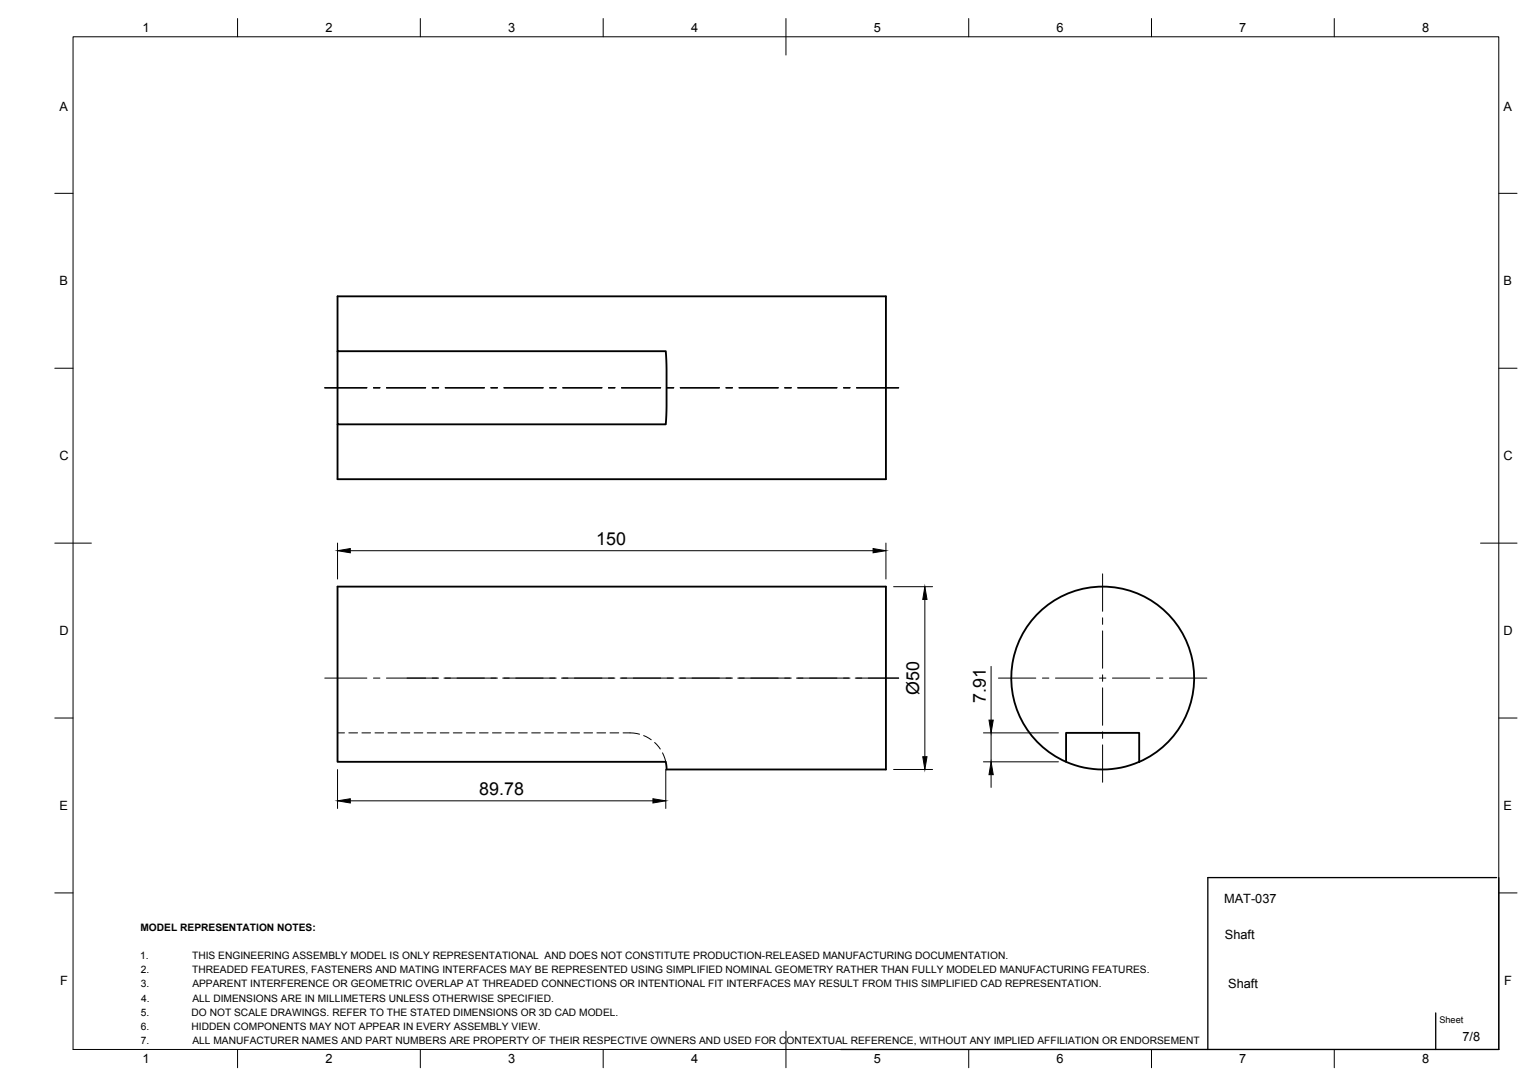
ISO-10303-21;
HEADER;
/* Generated by software containing ST-Developer
 * from STEP Tools, Inc. (www.steptools.com) 
 */

FILE_DESCRIPTION(
/* description */ ('STEP AP214'),
/* implementation_level */ '2;1');

FILE_NAME(
/* name */ 'shaft.step',
/* time_stamp */ '2026-11-14T21:09:07-08:00',
/* author */ (''),
/* organization */ (''),
/* preprocessor_version */ 'ST-DEVELOPER v20.2',
/* originating_system */ 'Autodesk Translation Framework v15.17.0.0',
/* authorisation */ '');

FILE_SCHEMA (('AUTOMOTIVE_DESIGN { 1 0 10303 214 3 1 1 }'));
ENDSEC;

DATA;
#10=MECHANICAL_DESIGN_GEOMETRIC_PRESENTATION_REPRESENTATION('',(#83),#2059);
#69=SHAPE_REPRESENTATION_RELATIONSHIP('SRR','None',#2099,#76);
#76=ADVANCED_BREP_SHAPE_REPRESENTATION('',(#90),#2057);
#83=STYLED_ITEM('',(#2142),#90);
#90=MANIFOLD_SOLID_BREP('Body1',#980);
#116=PLANE('',#1148);
#117=PLANE('',#1149);
#118=PLANE('',#1150);
#119=PLANE('',#1152);
#120=PLANE('',#1154);
#155=B_SPLINE_CURVE_WITH_KNOTS('',3,(#1969,#1970,#1971,#1972,#1973,#1974,
#1975,#1976,#1977,#1978,#1979,#1980,#1981,#1982),.UNSPECIFIED.,.F.,.F.,
(4,2,2,2,2,2,4),(-3.67157631505784,-3.33396300865433,-3.01698728047981,
-2.7000115523053,-2.38303582413079,-2.06606009595627,-1.72844678955265),
 .UNSPECIFIED.);
#199=FACE_OUTER_BOUND('',#275,.T.);
#200=FACE_OUTER_BOUND('',#276,.T.);
#201=FACE_OUTER_BOUND('',#277,.T.);
#202=FACE_OUTER_BOUND('',#278,.T.);
#203=FACE_OUTER_BOUND('',#279,.T.);
#204=FACE_OUTER_BOUND('',#280,.T.);
#205=FACE_OUTER_BOUND('',#281,.T.);
#275=EDGE_LOOP('',(#843,#844,#845,#846,#847,#848,#849,#850));
#276=EDGE_LOOP('',(#851,#852,#853,#854,#855));
#277=EDGE_LOOP('',(#856));
#278=EDGE_LOOP('',(#857,#858,#859,#860));
#279=EDGE_LOOP('',(#861,#862,#863,#864));
#280=EDGE_LOOP('',(#865,#866,#867,#868));
#281=EDGE_LOOP('',(#869,#870,#871,#872));
#336=LINE('',#1962,#401);
#337=LINE('',#1967,#402);
#338=LINE('',#1983,#403);
#339=LINE('',#1986,#404);
#340=LINE('',#1988,#405);
#341=LINE('',#1989,#406);
#342=LINE('',#1994,#407);
#343=LINE('',#1997,#408);
#344=LINE('',#2000,#409);
#401=VECTOR('',#1400,25.0000000000002);
#402=VECTOR('',#1405,1000.);
#403=VECTOR('',#1406,1000.);
#404=VECTOR('',#1409,1000.);
#405=VECTOR('',#1410,1000.);
#406=VECTOR('',#1411,1000.);
#407=VECTOR('',#1418,1000.);
#408=VECTOR('',#1421,1000.);
#409=VECTOR('',#1426,1000.);
#452=CIRCLE('',#1145,25.0000000000002);
#453=CIRCLE('',#1146,25.0000000000002);
#454=CIRCLE('',#1147,25.0000000000002);
#455=CIRCLE('',#1151,10.0000000000001);
#456=CIRCLE('',#1153,10.0000000000001);
#522=VERTEX_POINT('',#1958);
#523=VERTEX_POINT('',#1959);
#524=VERTEX_POINT('',#1961);
#525=VERTEX_POINT('',#1964);
#526=VERTEX_POINT('',#1966);
#527=VERTEX_POINT('',#1968);
#528=VERTEX_POINT('',#1985);
#529=VERTEX_POINT('',#1987);
#530=VERTEX_POINT('',#1992);
#531=VERTEX_POINT('',#1996);
#632=EDGE_CURVE('',#522,#523,#452,.T.);
#633=EDGE_CURVE('',#523,#524,#336,.T.);
#634=EDGE_CURVE('',#524,#524,#453,.T.);
#635=EDGE_CURVE('',#523,#525,#454,.T.);
#636=EDGE_CURVE('',#526,#525,#337,.T.);
#637=EDGE_CURVE('',#526,#527,#155,.T.);
#638=EDGE_CURVE('',#522,#527,#338,.T.);
#639=EDGE_CURVE('',#528,#522,#339,.T.);
#640=EDGE_CURVE('',#528,#529,#340,.T.);
#641=EDGE_CURVE('',#529,#525,#341,.T.);
#642=EDGE_CURVE('',#527,#530,#455,.T.);
#643=EDGE_CURVE('',#530,#528,#342,.T.);
#644=EDGE_CURVE('',#531,#529,#343,.T.);
#645=EDGE_CURVE('',#531,#526,#456,.T.);
#646=EDGE_CURVE('',#530,#531,#344,.T.);
#843=ORIENTED_EDGE('',*,*,#632,.T.);
#844=ORIENTED_EDGE('',*,*,#633,.T.);
#845=ORIENTED_EDGE('',*,*,#634,.F.);
#846=ORIENTED_EDGE('',*,*,#633,.F.);
#847=ORIENTED_EDGE('',*,*,#635,.T.);
#848=ORIENTED_EDGE('',*,*,#636,.F.);
#849=ORIENTED_EDGE('',*,*,#637,.T.);
#850=ORIENTED_EDGE('',*,*,#638,.F.);
#851=ORIENTED_EDGE('',*,*,#639,.F.);
#852=ORIENTED_EDGE('',*,*,#640,.T.);
#853=ORIENTED_EDGE('',*,*,#641,.T.);
#854=ORIENTED_EDGE('',*,*,#635,.F.);
#855=ORIENTED_EDGE('',*,*,#632,.F.);
#856=ORIENTED_EDGE('',*,*,#634,.T.);
#857=ORIENTED_EDGE('',*,*,#638,.T.);
#858=ORIENTED_EDGE('',*,*,#642,.T.);
#859=ORIENTED_EDGE('',*,*,#643,.T.);
#860=ORIENTED_EDGE('',*,*,#639,.T.);
#861=ORIENTED_EDGE('',*,*,#644,.F.);
#862=ORIENTED_EDGE('',*,*,#645,.T.);
#863=ORIENTED_EDGE('',*,*,#636,.T.);
#864=ORIENTED_EDGE('',*,*,#641,.F.);
#865=ORIENTED_EDGE('',*,*,#643,.F.);
#866=ORIENTED_EDGE('',*,*,#646,.T.);
#867=ORIENTED_EDGE('',*,*,#644,.T.);
#868=ORIENTED_EDGE('',*,*,#640,.F.);
#869=ORIENTED_EDGE('',*,*,#642,.F.);
#870=ORIENTED_EDGE('',*,*,#637,.F.);
#871=ORIENTED_EDGE('',*,*,#645,.F.);
#872=ORIENTED_EDGE('',*,*,#646,.F.);
#915=CYLINDRICAL_SURFACE('',#1144,25.0000000000002);
#916=CYLINDRICAL_SURFACE('',#1155,10.0000000000001);
#962=ADVANCED_FACE('',(#199),#915,.T.);
#963=ADVANCED_FACE('',(#200),#116,.F.);
#964=ADVANCED_FACE('',(#201),#117,.T.);
#965=ADVANCED_FACE('',(#202),#118,.T.);
#966=ADVANCED_FACE('',(#203),#119,.T.);
#967=ADVANCED_FACE('',(#204),#120,.T.);
#968=ADVANCED_FACE('',(#205),#916,.F.);
#980=CLOSED_SHELL('',(#962,#963,#964,#965,#966,#967,#968));
#1143=AXIS2_PLACEMENT_3D('',#1956,#1394,#1395);
#1144=AXIS2_PLACEMENT_3D('',#1957,#1396,#1397);
#1145=AXIS2_PLACEMENT_3D('',#1960,#1398,#1399);
#1146=AXIS2_PLACEMENT_3D('',#1963,#1401,#1402);
#1147=AXIS2_PLACEMENT_3D('',#1965,#1403,#1404);
#1148=AXIS2_PLACEMENT_3D('',#1984,#1407,#1408);
#1149=AXIS2_PLACEMENT_3D('',#1990,#1412,#1413);
#1150=AXIS2_PLACEMENT_3D('',#1991,#1414,#1415);
#1151=AXIS2_PLACEMENT_3D('',#1993,#1416,#1417);
#1152=AXIS2_PLACEMENT_3D('',#1995,#1419,#1420);
#1153=AXIS2_PLACEMENT_3D('',#1998,#1422,#1423);
#1154=AXIS2_PLACEMENT_3D('',#1999,#1424,#1425);
#1155=AXIS2_PLACEMENT_3D('',#2001,#1427,#1428);
#1394=DIRECTION('axis',(0.,0.,1.));
#1395=DIRECTION('refdir',(1.,0.,0.));
#1396=DIRECTION('center_axis',(1.40946282423116E-17,-7.79000143905744E-30,
-1.));
#1397=DIRECTION('ref_axis',(-1.,1.65167752030648E-30,-1.40946282423116E-17));
#1398=DIRECTION('center_axis',(-1.40946282423116E-17,7.79000143905744E-30,
1.));
#1399=DIRECTION('ref_axis',(1.,-1.65167752030648E-30,1.40946282423116E-17));
#1400=DIRECTION('',(-1.40946282423116E-17,7.79000143905744E-30,1.));
#1401=DIRECTION('center_axis',(-1.40946282423116E-17,7.79000143905744E-30,
1.));
#1402=DIRECTION('ref_axis',(1.,-1.65167752030648E-30,1.40946282423116E-17));
#1403=DIRECTION('center_axis',(-1.40946282423116E-17,7.79000143905744E-30,
1.));
#1404=DIRECTION('ref_axis',(1.,-1.65167752030648E-30,1.40946282423116E-17));
#1405=DIRECTION('',(1.40946282423116E-17,-7.79000143905744E-30,-1.));
#1406=DIRECTION('',(-1.40946282423116E-17,7.79000143905744E-30,1.));
#1407=DIRECTION('center_axis',(-1.40946282423114E-17,7.79000143905744E-30,
1.));
#1408=DIRECTION('ref_axis',(1.,-1.65167752030648E-30,1.40946282423114E-17));
#1409=DIRECTION('',(-1.84889274661175E-30,1.,7.29696337329436E-30));
#1410=DIRECTION('',(1.,-1.65167752030648E-30,1.40946282423114E-17));
#1411=DIRECTION('',(-1.84889274661175E-30,1.,7.29696337329436E-30));
#1412=DIRECTION('center_axis',(-1.40946282423114E-17,7.79000143905744E-30,
1.));
#1413=DIRECTION('ref_axis',(1.,-1.65167752030648E-30,1.40946282423114E-17));
#1414=DIRECTION('center_axis',(1.,-1.7009813268828E-30,1.40946282423116E-17));
#1415=DIRECTION('ref_axis',(1.40946282423116E-17,-7.79000143905744E-30,
-1.));
#1416=DIRECTION('center_axis',(1.,-1.7009813268828E-30,1.04083408558607E-17));
#1417=DIRECTION('ref_axis',(1.04083408558607E-17,-1.77043934396503E-47,
-1.));
#1418=DIRECTION('',(1.04083408558609E-17,-7.69139382590482E-30,-1.));
#1419=DIRECTION('center_axis',(-1.,1.7009813268828E-30,-1.40946282423116E-17));
#1420=DIRECTION('ref_axis',(-1.40946282423116E-17,7.79000143905744E-30,
1.));
#1421=DIRECTION('',(1.04083408558609E-17,-7.69139382590482E-30,-1.));
#1422=DIRECTION('center_axis',(-1.,1.7009813268828E-30,-1.04083408558607E-17));
#1423=DIRECTION('ref_axis',(-1.04083408558607E-17,1.77043934396503E-47,
1.));
#1424=DIRECTION('center_axis',(-1.84889274661175E-30,1.,-7.79000143905744E-30));
#1425=DIRECTION('ref_axis',(-1.40946282423116E-17,7.79000143905744E-30,
1.));
#1426=DIRECTION('',(1.,-1.65167752030648E-30,1.40946282423114E-17));
#1427=DIRECTION('center_axis',(1.,-1.65167752030648E-30,1.40946282423114E-17));
#1428=DIRECTION('ref_axis',(1.40946282423114E-17,-2.32797806249026E-47,
-1.));
#1956=CARTESIAN_POINT('',(0.,0.,0.));
#1957=CARTESIAN_POINT('Origin',(-2.22044604925031E-13,0.,150.));
#1958=CARTESIAN_POINT('',(-10.0000000000013,22.9128784747792,-8.88178419700125E-13));
#1959=CARTESIAN_POINT('',(24.9999999999999,-3.06161699786961E-15,-8.88178419700125E-13));
#1960=CARTESIAN_POINT('Origin',(0.,0.,0.));
#1961=CARTESIAN_POINT('',(24.9999999999999,-3.06161699786845E-15,150.));
#1962=CARTESIAN_POINT('',(24.9999999999999,-3.06161699786845E-15,150.));
#1963=CARTESIAN_POINT('Origin',(-2.22044604925031E-13,0.,150.));
#1964=CARTESIAN_POINT('',(10.,22.9128784747792,0.));
#1965=CARTESIAN_POINT('Origin',(0.,0.,0.));
#1966=CARTESIAN_POINT('',(9.99999999999912,22.9128784747793,89.7797711496207));
#1967=CARTESIAN_POINT('',(9.99999999999979,22.9128784747792,150.));
#1968=CARTESIAN_POINT('',(-10.000000000001,22.9128784747793,89.7797711496216));
#1969=CARTESIAN_POINT('Ctrl Pts',(9.99999999999965,22.9128784747794,89.7797711496257));
#1970=CARTESIAN_POINT('Ctrl Pts',(8.91671999216883,23.3856606304668,89.8806685836023));
#1971=CARTESIAN_POINT('Ctrl Pts',(7.77197604014579,23.792186686818,89.9320009552562));
#1972=CARTESIAN_POINT('Ctrl Pts',(5.50330393661502,24.4133362342407,89.9873423916812));
#1973=CARTESIAN_POINT('Ctrl Pts',(4.3815649951061,24.6385720078244,89.9945429930909));
#1974=CARTESIAN_POINT('Ctrl Pts',(2.15820493465309,24.9318971171076,90.0008440556194));
#1975=CARTESIAN_POINT('Ctrl Pts',(1.05658576058149,25.0000000000002,90.0000000000046));
#1976=CARTESIAN_POINT('Ctrl Pts',(-1.05658576058194,25.0000000000002,90.0000000000046));
#1977=CARTESIAN_POINT('Ctrl Pts',(-2.15820493465353,24.9318971171076,90.0008440556194));
#1978=CARTESIAN_POINT('Ctrl Pts',(-4.38156499510654,24.6385720078244,89.9945429930909));
#1979=CARTESIAN_POINT('Ctrl Pts',(-5.50330393661546,24.4133362342407,89.9873423916812));
#1980=CARTESIAN_POINT('Ctrl Pts',(-7.77197604014664,23.7921866868179,89.9320009552562));
#1981=CARTESIAN_POINT('Ctrl Pts',(-8.91671999217008,23.3856606304665,89.8806685836023));
#1982=CARTESIAN_POINT('Ctrl Pts',(-10.0000000000012,22.9128784747789,89.7797711496256));
#1983=CARTESIAN_POINT('',(-10.,22.9128784747792,150.));
#1984=CARTESIAN_POINT('Origin',(0.,0.,0.));
#1985=CARTESIAN_POINT('',(-10.0000000000013,15.,-8.88178419700125E-13));
#1986=CARTESIAN_POINT('',(-10.0000000000013,0.,-8.88178419700125E-13));
#1987=CARTESIAN_POINT('',(10.,15.,0.));
#1988=CARTESIAN_POINT('',(-10.0000000000013,15.,-8.88178419700125E-13));
#1989=CARTESIAN_POINT('',(10.,15.,0.));
#1990=CARTESIAN_POINT('Origin',(-2.22044604925031E-13,0.,150.));
#1991=CARTESIAN_POINT('Origin',(-10.0000000000002,27.1241010986052,90.0000000000003));
#1992=CARTESIAN_POINT('',(-10.0000000000009,15.0000000000003,80.0000000000041));
#1993=CARTESIAN_POINT('Origin',(-10.000000000001,25.,80.0000000000045));
#1994=CARTESIAN_POINT('',(-10.0000000000002,15.,90.0000000000003));
#1995=CARTESIAN_POINT('Origin',(9.99999999999979,15.,89.9999999999994));
#1996=CARTESIAN_POINT('',(9.99999999999945,15.,80.0000000000036));
#1997=CARTESIAN_POINT('',(9.99999999999979,15.,89.9999999999994));
#1998=CARTESIAN_POINT('Origin',(9.99999999999934,25.,80.0000000000036));
#1999=CARTESIAN_POINT('Origin',(-10.0000000000002,15.,90.0000000000003));
#2000=CARTESIAN_POINT('',(-10.0000000000009,15.0000000000003,80.0000000000041));
#2001=CARTESIAN_POINT('Origin',(-10.000000000001,25.,80.0000000000045));
#2048=UNCERTAINTY_MEASURE_WITH_UNIT(LENGTH_MEASURE(0.01),#2060,
'DISTANCE_ACCURACY_VALUE',
'Maximum model space distance between geometric entities at asserted c
onnectivities');
#2050=UNCERTAINTY_MEASURE_WITH_UNIT(LENGTH_MEASURE(0.01),#2060,
'DISTANCE_ACCURACY_VALUE',
'Maximum model space distance between geometric entities at asserted c
onnectivities');
#2057=(
GEOMETRIC_REPRESENTATION_CONTEXT(3)
GLOBAL_UNCERTAINTY_ASSIGNED_CONTEXT((#2048))
GLOBAL_UNIT_ASSIGNED_CONTEXT((#2060,#2062,#2063))
REPRESENTATION_CONTEXT('','3D')
);
#2059=(
GEOMETRIC_REPRESENTATION_CONTEXT(3)
GLOBAL_UNCERTAINTY_ASSIGNED_CONTEXT((#2050))
GLOBAL_UNIT_ASSIGNED_CONTEXT((#2060,#2062,#2063))
REPRESENTATION_CONTEXT('','3D')
);
#2060=(
LENGTH_UNIT()
NAMED_UNIT(*)
SI_UNIT(.MILLI.,.METRE.)
);
#2062=(
NAMED_UNIT(*)
PLANE_ANGLE_UNIT()
SI_UNIT($,.RADIAN.)
);
#2063=(
NAMED_UNIT(*)
SI_UNIT($,.STERADIAN.)
SOLID_ANGLE_UNIT()
);
#2070=SHAPE_DEFINITION_REPRESENTATION(#2078,#2099);
#2078=PRODUCT_DEFINITION_SHAPE('',$,#2108);
#2099=SHAPE_REPRESENTATION('',(#1143),#2057);
#2101=PRODUCT_DEFINITION_CONTEXT('part definition',#2127,'design');
#2108=PRODUCT_DEFINITION('Shaft','shaft',#2116,#2101);
#2116=PRODUCT_DEFINITION_FORMATION('',$,#2135);
#2127=APPLICATION_CONTEXT(
'Core Data for Automotive Mechanical Design Process');
#2128=PRODUCT_CONTEXT('part definition',#2127,'mechanical');
#2135=PRODUCT('Shaft','shaft','Shaft',(#2128));
#2142=PRESENTATION_STYLE_ASSIGNMENT((#2148));
#2148=SURFACE_STYLE_USAGE(.BOTH.,#2154);
#2154=SURFACE_SIDE_STYLE('',(#2160));
#2160=SURFACE_STYLE_FILL_AREA(#2166);
#2166=FILL_AREA_STYLE('Opaque(122,133,145)',(#2172));
#2172=FILL_AREA_STYLE_COLOUR('Opaque(122,133,145)',#2178);
#2178=COLOUR_RGB('Opaque(122,133,145)',0.47843137254902,0.52156862745098,
0.568627450980392);
ENDSEC;
END-ISO-10303-21;
